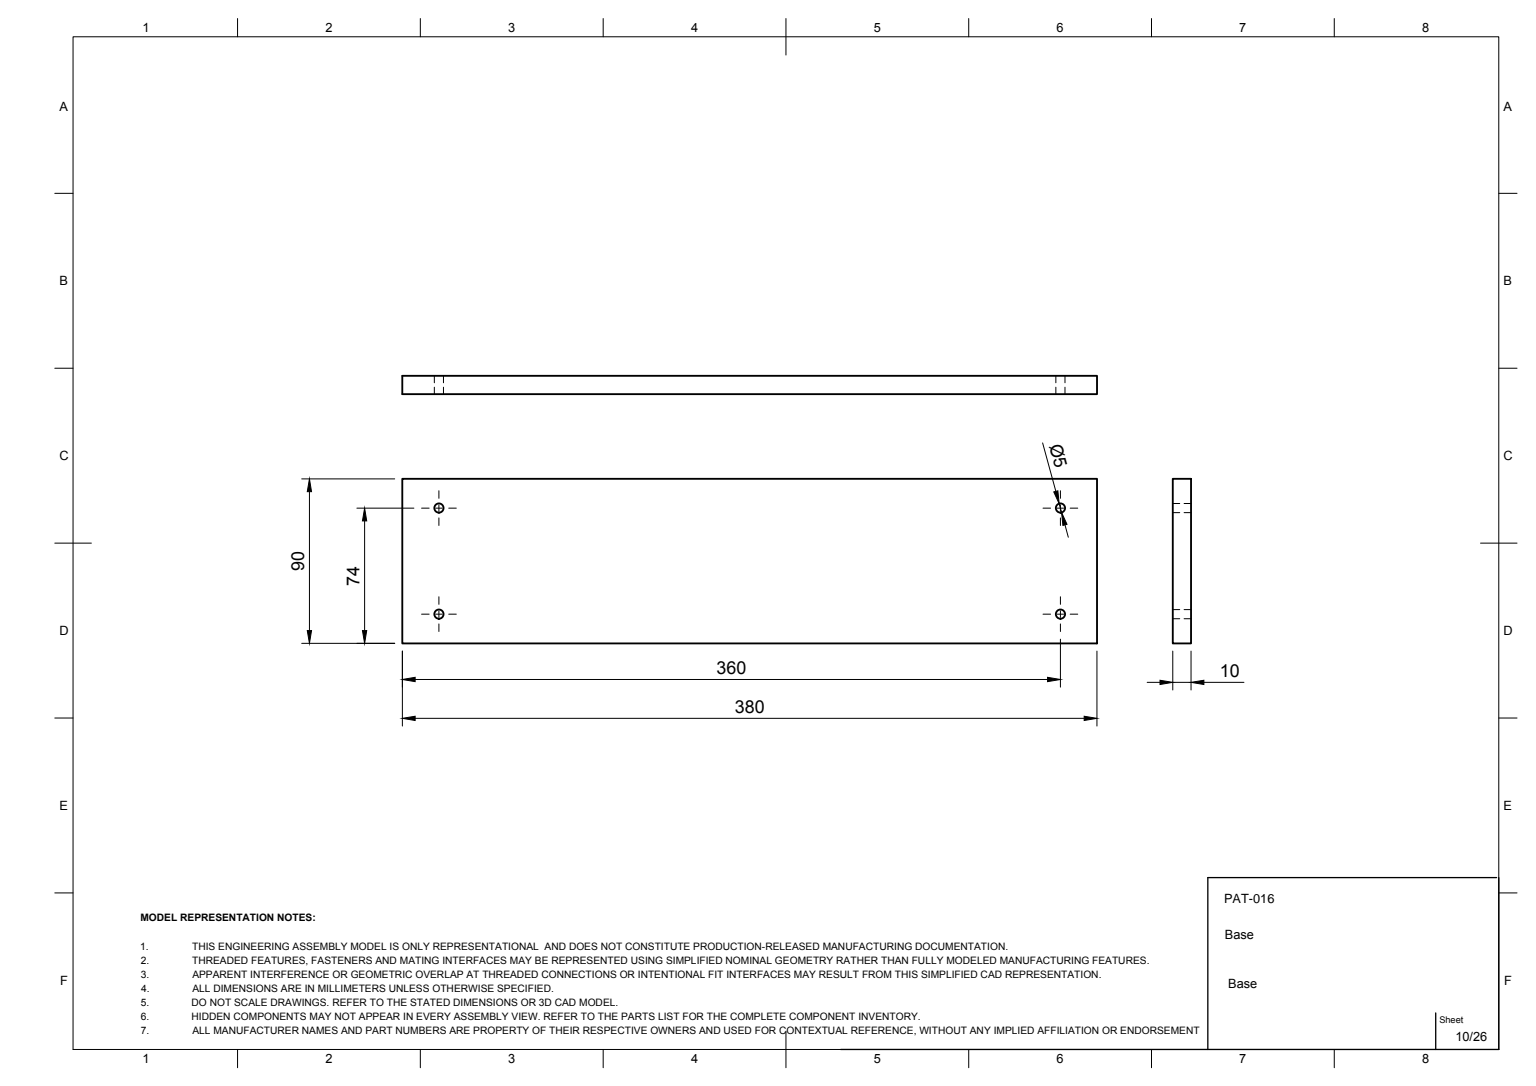
ISO-10303-21;
HEADER;
/* Generated by software containing ST-Developer
 * from STEP Tools, Inc. (www.steptools.com) 
 */

FILE_DESCRIPTION(
/* description */ ('Bracket-mounted idler roller'),
/* implementation_level */ '2;1');

FILE_NAME(
/* name */ 'Base.step',
/* time_stamp */ '2026-10-28T03:26:42-07:00',
/* author */ (''),
/* organization */ (''),
/* preprocessor_version */ 'ST-DEVELOPER v20.2',
/* originating_system */ 'Autodesk Translation Framework v15.17.0.0',
/* authorisation */ '');

FILE_SCHEMA (('AUTOMOTIVE_DESIGN { 1 0 10303 214 3 1 1 }'));
ENDSEC;

DATA;
#10=MECHANICAL_DESIGN_GEOMETRIC_PRESENTATION_REPRESENTATION('',(#285),#6241);
#243=SHAPE_REPRESENTATION_RELATIONSHIP('SRR','None',#6347,#264);
#264=ADVANCED_BREP_SHAPE_REPRESENTATION('',(#314),#6223);
#285=STYLED_ITEM('',(#6517),#314);
#314=MANIFOLD_SOLID_BREP('Body1',#3187);
#358=FACE_BOUND('',#785,.T.);
#359=FACE_BOUND('',#786,.T.);
#360=FACE_BOUND('',#787,.T.);
#361=FACE_BOUND('',#788,.T.);
#362=FACE_BOUND('',#790,.T.);
#363=FACE_BOUND('',#791,.T.);
#364=FACE_BOUND('',#792,.T.);
#365=FACE_BOUND('',#793,.T.);
#449=PLANE('',#3542);
#450=PLANE('',#3543);
#451=PLANE('',#3544);
#452=PLANE('',#3545);
#453=PLANE('',#3546);
#454=PLANE('',#3547);
#563=FACE_OUTER_BOUND('',#776,.T.);
#564=FACE_OUTER_BOUND('',#777,.T.);
#565=FACE_OUTER_BOUND('',#778,.T.);
#566=FACE_OUTER_BOUND('',#779,.T.);
#567=FACE_OUTER_BOUND('',#780,.T.);
#568=FACE_OUTER_BOUND('',#781,.T.);
#569=FACE_OUTER_BOUND('',#782,.T.);
#570=FACE_OUTER_BOUND('',#783,.T.);
#571=FACE_OUTER_BOUND('',#784,.T.);
#572=FACE_OUTER_BOUND('',#789,.T.);
#776=EDGE_LOOP('',(#2352,#2353,#2354,#2355));
#777=EDGE_LOOP('',(#2356,#2357,#2358,#2359));
#778=EDGE_LOOP('',(#2360,#2361,#2362,#2363));
#779=EDGE_LOOP('',(#2364,#2365,#2366,#2367));
#780=EDGE_LOOP('',(#2368,#2369,#2370,#2371));
#781=EDGE_LOOP('',(#2372,#2373,#2374,#2375));
#782=EDGE_LOOP('',(#2376,#2377,#2378,#2379));
#783=EDGE_LOOP('',(#2380,#2381,#2382,#2383));
#784=EDGE_LOOP('',(#2384,#2385,#2386,#2387));
#785=EDGE_LOOP('',(#2388));
#786=EDGE_LOOP('',(#2389));
#787=EDGE_LOOP('',(#2390));
#788=EDGE_LOOP('',(#2391));
#789=EDGE_LOOP('',(#2392,#2393,#2394,#2395));
#790=EDGE_LOOP('',(#2396));
#791=EDGE_LOOP('',(#2397));
#792=EDGE_LOOP('',(#2398));
#793=EDGE_LOOP('',(#2399));
#1042=LINE('',#5164,#1224);
#1043=LINE('',#5170,#1225);
#1044=LINE('',#5176,#1226);
#1045=LINE('',#5182,#1227);
#1046=LINE('',#5187,#1228);
#1047=LINE('',#5189,#1229);
#1048=LINE('',#5191,#1230);
#1049=LINE('',#5192,#1231);
#1050=LINE('',#5195,#1232);
#1051=LINE('',#5197,#1233);
#1052=LINE('',#5198,#1234);
#1053=LINE('',#5201,#1235);
#1054=LINE('',#5203,#1236);
#1055=LINE('',#5204,#1237);
#1056=LINE('',#5206,#1238);
#1057=LINE('',#5207,#1239);
#1224=VECTOR('',#4123,0.25);
#1225=VECTOR('',#4130,0.25);
#1226=VECTOR('',#4137,0.25);
#1227=VECTOR('',#4144,0.25);
#1228=VECTOR('',#4149,1.);
#1229=VECTOR('',#4150,1.);
#1230=VECTOR('',#4151,1.);
#1231=VECTOR('',#4152,1.);
#1232=VECTOR('',#4155,1.);
#1233=VECTOR('',#4156,1.);
#1234=VECTOR('',#4157,1.);
#1235=VECTOR('',#4160,1.);
#1236=VECTOR('',#4161,1.);
#1237=VECTOR('',#4162,1.);
#1238=VECTOR('',#4165,1.);
#1239=VECTOR('',#4166,1.);
#1373=CIRCLE('',#3531,0.25);
#1374=CIRCLE('',#3532,0.25);
#1375=CIRCLE('',#3534,0.25);
#1376=CIRCLE('',#3535,0.25);
#1377=CIRCLE('',#3537,0.25);
#1378=CIRCLE('',#3538,0.25);
#1379=CIRCLE('',#3540,0.25);
#1380=CIRCLE('',#3541,0.25);
#1586=VERTEX_POINT('',#5161);
#1587=VERTEX_POINT('',#5163);
#1588=VERTEX_POINT('',#5167);
#1589=VERTEX_POINT('',#5169);
#1590=VERTEX_POINT('',#5173);
#1591=VERTEX_POINT('',#5175);
#1592=VERTEX_POINT('',#5179);
#1593=VERTEX_POINT('',#5181);
#1594=VERTEX_POINT('',#5185);
#1595=VERTEX_POINT('',#5186);
#1596=VERTEX_POINT('',#5188);
#1597=VERTEX_POINT('',#5190);
#1598=VERTEX_POINT('',#5194);
#1599=VERTEX_POINT('',#5196);
#1600=VERTEX_POINT('',#5200);
#1601=VERTEX_POINT('',#5202);
#1878=EDGE_CURVE('',#1586,#1586,#1373,.T.);
#1879=EDGE_CURVE('',#1586,#1587,#1042,.T.);
#1880=EDGE_CURVE('',#1587,#1587,#1374,.T.);
#1881=EDGE_CURVE('',#1588,#1588,#1375,.T.);
#1882=EDGE_CURVE('',#1588,#1589,#1043,.T.);
#1883=EDGE_CURVE('',#1589,#1589,#1376,.T.);
#1884=EDGE_CURVE('',#1590,#1590,#1377,.T.);
#1885=EDGE_CURVE('',#1590,#1591,#1044,.T.);
#1886=EDGE_CURVE('',#1591,#1591,#1378,.T.);
#1887=EDGE_CURVE('',#1592,#1592,#1379,.T.);
#1888=EDGE_CURVE('',#1592,#1593,#1045,.T.);
#1889=EDGE_CURVE('',#1593,#1593,#1380,.T.);
#1890=EDGE_CURVE('',#1594,#1595,#1046,.T.);
#1891=EDGE_CURVE('',#1595,#1596,#1047,.T.);
#1892=EDGE_CURVE('',#1597,#1596,#1048,.T.);
#1893=EDGE_CURVE('',#1594,#1597,#1049,.T.);
#1894=EDGE_CURVE('',#1598,#1594,#1050,.T.);
#1895=EDGE_CURVE('',#1599,#1597,#1051,.T.);
#1896=EDGE_CURVE('',#1598,#1599,#1052,.T.);
#1897=EDGE_CURVE('',#1600,#1598,#1053,.T.);
#1898=EDGE_CURVE('',#1601,#1599,#1054,.T.);
#1899=EDGE_CURVE('',#1600,#1601,#1055,.T.);
#1900=EDGE_CURVE('',#1595,#1600,#1056,.T.);
#1901=EDGE_CURVE('',#1596,#1601,#1057,.T.);
#2352=ORIENTED_EDGE('',*,*,#1878,.F.);
#2353=ORIENTED_EDGE('',*,*,#1879,.T.);
#2354=ORIENTED_EDGE('',*,*,#1880,.F.);
#2355=ORIENTED_EDGE('',*,*,#1879,.F.);
#2356=ORIENTED_EDGE('',*,*,#1881,.F.);
#2357=ORIENTED_EDGE('',*,*,#1882,.T.);
#2358=ORIENTED_EDGE('',*,*,#1883,.F.);
#2359=ORIENTED_EDGE('',*,*,#1882,.F.);
#2360=ORIENTED_EDGE('',*,*,#1884,.F.);
#2361=ORIENTED_EDGE('',*,*,#1885,.T.);
#2362=ORIENTED_EDGE('',*,*,#1886,.F.);
#2363=ORIENTED_EDGE('',*,*,#1885,.F.);
#2364=ORIENTED_EDGE('',*,*,#1887,.F.);
#2365=ORIENTED_EDGE('',*,*,#1888,.T.);
#2366=ORIENTED_EDGE('',*,*,#1889,.F.);
#2367=ORIENTED_EDGE('',*,*,#1888,.F.);
#2368=ORIENTED_EDGE('',*,*,#1890,.T.);
#2369=ORIENTED_EDGE('',*,*,#1891,.T.);
#2370=ORIENTED_EDGE('',*,*,#1892,.F.);
#2371=ORIENTED_EDGE('',*,*,#1893,.F.);
#2372=ORIENTED_EDGE('',*,*,#1894,.T.);
#2373=ORIENTED_EDGE('',*,*,#1893,.T.);
#2374=ORIENTED_EDGE('',*,*,#1895,.F.);
#2375=ORIENTED_EDGE('',*,*,#1896,.F.);
#2376=ORIENTED_EDGE('',*,*,#1897,.T.);
#2377=ORIENTED_EDGE('',*,*,#1896,.T.);
#2378=ORIENTED_EDGE('',*,*,#1898,.F.);
#2379=ORIENTED_EDGE('',*,*,#1899,.F.);
#2380=ORIENTED_EDGE('',*,*,#1900,.T.);
#2381=ORIENTED_EDGE('',*,*,#1899,.T.);
#2382=ORIENTED_EDGE('',*,*,#1901,.F.);
#2383=ORIENTED_EDGE('',*,*,#1891,.F.);
#2384=ORIENTED_EDGE('',*,*,#1901,.T.);
#2385=ORIENTED_EDGE('',*,*,#1898,.T.);
#2386=ORIENTED_EDGE('',*,*,#1895,.T.);
#2387=ORIENTED_EDGE('',*,*,#1892,.T.);
#2388=ORIENTED_EDGE('',*,*,#1880,.T.);
#2389=ORIENTED_EDGE('',*,*,#1883,.T.);
#2390=ORIENTED_EDGE('',*,*,#1886,.T.);
#2391=ORIENTED_EDGE('',*,*,#1889,.T.);
#2392=ORIENTED_EDGE('',*,*,#1900,.F.);
#2393=ORIENTED_EDGE('',*,*,#1890,.F.);
#2394=ORIENTED_EDGE('',*,*,#1894,.F.);
#2395=ORIENTED_EDGE('',*,*,#1897,.F.);
#2396=ORIENTED_EDGE('',*,*,#1878,.T.);
#2397=ORIENTED_EDGE('',*,*,#1881,.T.);
#2398=ORIENTED_EDGE('',*,*,#1884,.T.);
#2399=ORIENTED_EDGE('',*,*,#1887,.T.);
#2943=CYLINDRICAL_SURFACE('',#3530,0.25);
#2944=CYLINDRICAL_SURFACE('',#3533,0.25);
#2945=CYLINDRICAL_SURFACE('',#3536,0.25);
#2946=CYLINDRICAL_SURFACE('',#3539,0.25);
#3038=ADVANCED_FACE('',(#563),#2943,.F.);
#3039=ADVANCED_FACE('',(#564),#2944,.F.);
#3040=ADVANCED_FACE('',(#565),#2945,.F.);
#3041=ADVANCED_FACE('',(#566),#2946,.F.);
#3042=ADVANCED_FACE('',(#567),#449,.T.);
#3043=ADVANCED_FACE('',(#568),#450,.T.);
#3044=ADVANCED_FACE('',(#569),#451,.T.);
#3045=ADVANCED_FACE('',(#570),#452,.T.);
#3046=ADVANCED_FACE('',(#571,#358,#359,#360,#361),#453,.T.);
#3047=ADVANCED_FACE('',(#572,#362,#363,#364,#365),#454,.F.);
#3187=CLOSED_SHELL('',(#3038,#3039,#3040,#3041,#3042,#3043,#3044,#3045,
#3046,#3047));
#3529=AXIS2_PLACEMENT_3D('',#5159,#4117,#4118);
#3530=AXIS2_PLACEMENT_3D('',#5160,#4119,#4120);
#3531=AXIS2_PLACEMENT_3D('',#5162,#4121,#4122);
#3532=AXIS2_PLACEMENT_3D('',#5165,#4124,#4125);
#3533=AXIS2_PLACEMENT_3D('',#5166,#4126,#4127);
#3534=AXIS2_PLACEMENT_3D('',#5168,#4128,#4129);
#3535=AXIS2_PLACEMENT_3D('',#5171,#4131,#4132);
#3536=AXIS2_PLACEMENT_3D('',#5172,#4133,#4134);
#3537=AXIS2_PLACEMENT_3D('',#5174,#4135,#4136);
#3538=AXIS2_PLACEMENT_3D('',#5177,#4138,#4139);
#3539=AXIS2_PLACEMENT_3D('',#5178,#4140,#4141);
#3540=AXIS2_PLACEMENT_3D('',#5180,#4142,#4143);
#3541=AXIS2_PLACEMENT_3D('',#5183,#4145,#4146);
#3542=AXIS2_PLACEMENT_3D('',#5184,#4147,#4148);
#3543=AXIS2_PLACEMENT_3D('',#5193,#4153,#4154);
#3544=AXIS2_PLACEMENT_3D('',#5199,#4158,#4159);
#3545=AXIS2_PLACEMENT_3D('',#5205,#4163,#4164);
#3546=AXIS2_PLACEMENT_3D('',#5208,#4167,#4168);
#3547=AXIS2_PLACEMENT_3D('',#5209,#4169,#4170);
#4117=DIRECTION('axis',(0.,0.,1.));
#4118=DIRECTION('refdir',(1.,0.,0.));
#4119=DIRECTION('center_axis',(0.,0.,1.));
#4120=DIRECTION('ref_axis',(1.,0.,0.));
#4121=DIRECTION('center_axis',(0.,0.,1.));
#4122=DIRECTION('ref_axis',(1.,0.,0.));
#4123=DIRECTION('',(0.,0.,1.));
#4124=DIRECTION('center_axis',(0.,0.,-1.));
#4125=DIRECTION('ref_axis',(1.,0.,0.));
#4126=DIRECTION('center_axis',(0.,0.,1.));
#4127=DIRECTION('ref_axis',(1.,0.,0.));
#4128=DIRECTION('center_axis',(0.,0.,1.));
#4129=DIRECTION('ref_axis',(1.,0.,0.));
#4130=DIRECTION('',(0.,0.,1.));
#4131=DIRECTION('center_axis',(0.,0.,-1.));
#4132=DIRECTION('ref_axis',(1.,0.,0.));
#4133=DIRECTION('center_axis',(0.,0.,1.));
#4134=DIRECTION('ref_axis',(1.,0.,0.));
#4135=DIRECTION('center_axis',(0.,0.,1.));
#4136=DIRECTION('ref_axis',(1.,0.,0.));
#4137=DIRECTION('',(0.,0.,1.));
#4138=DIRECTION('center_axis',(0.,0.,-1.));
#4139=DIRECTION('ref_axis',(1.,0.,0.));
#4140=DIRECTION('center_axis',(0.,0.,1.));
#4141=DIRECTION('ref_axis',(1.,0.,0.));
#4142=DIRECTION('center_axis',(0.,0.,1.));
#4143=DIRECTION('ref_axis',(1.,0.,0.));
#4144=DIRECTION('',(0.,0.,1.));
#4145=DIRECTION('center_axis',(0.,0.,-1.));
#4146=DIRECTION('ref_axis',(1.,0.,0.));
#4147=DIRECTION('center_axis',(0.,1.,0.));
#4148=DIRECTION('ref_axis',(-1.,0.,0.));
#4149=DIRECTION('',(-1.,0.,0.));
#4150=DIRECTION('',(0.,0.,1.));
#4151=DIRECTION('',(-1.,0.,0.));
#4152=DIRECTION('',(0.,0.,1.));
#4153=DIRECTION('center_axis',(1.,0.,0.));
#4154=DIRECTION('ref_axis',(0.,1.,0.));
#4155=DIRECTION('',(0.,1.,0.));
#4156=DIRECTION('',(0.,1.,0.));
#4157=DIRECTION('',(0.,0.,1.));
#4158=DIRECTION('center_axis',(0.,-1.,0.));
#4159=DIRECTION('ref_axis',(1.,0.,0.));
#4160=DIRECTION('',(1.,0.,0.));
#4161=DIRECTION('',(1.,0.,0.));
#4162=DIRECTION('',(0.,0.,1.));
#4163=DIRECTION('center_axis',(-1.,0.,0.));
#4164=DIRECTION('ref_axis',(0.,-1.,0.));
#4165=DIRECTION('',(0.,-1.,0.));
#4166=DIRECTION('',(0.,-1.,0.));
#4167=DIRECTION('center_axis',(0.,0.,1.));
#4168=DIRECTION('ref_axis',(1.,0.,0.));
#4169=DIRECTION('center_axis',(0.,0.,1.));
#4170=DIRECTION('ref_axis',(1.,0.,0.));
#5159=CARTESIAN_POINT('',(0.,0.,0.));
#5160=CARTESIAN_POINT('Origin',(2.9,-2.,-0.1));
#5161=CARTESIAN_POINT('',(2.65,-2.,0.));
#5162=CARTESIAN_POINT('Origin',(2.9,-2.,0.));
#5163=CARTESIAN_POINT('',(2.65,-2.,1.));
#5164=CARTESIAN_POINT('',(2.65,-2.,-0.1));
#5165=CARTESIAN_POINT('Origin',(2.9,-2.,1.));
#5166=CARTESIAN_POINT('Origin',(-2.9,32.,-0.1));
#5167=CARTESIAN_POINT('',(-3.15,32.,0.));
#5168=CARTESIAN_POINT('Origin',(-2.9,32.,0.));
#5169=CARTESIAN_POINT('',(-3.15,32.,1.));
#5170=CARTESIAN_POINT('',(-3.15,32.,-0.1));
#5171=CARTESIAN_POINT('Origin',(-2.9,32.,1.));
#5172=CARTESIAN_POINT('Origin',(-2.9,-2.,-0.1));
#5173=CARTESIAN_POINT('',(-3.15,-2.,0.));
#5174=CARTESIAN_POINT('Origin',(-2.9,-2.,0.));
#5175=CARTESIAN_POINT('',(-3.15,-2.,1.));
#5176=CARTESIAN_POINT('',(-3.15,-2.,-0.1));
#5177=CARTESIAN_POINT('Origin',(-2.9,-2.,1.));
#5178=CARTESIAN_POINT('Origin',(2.9,32.,-0.1));
#5179=CARTESIAN_POINT('',(2.65,32.,0.));
#5180=CARTESIAN_POINT('Origin',(2.9,32.,0.));
#5181=CARTESIAN_POINT('',(2.65,32.,1.));
#5182=CARTESIAN_POINT('',(2.65,32.,-0.1));
#5183=CARTESIAN_POINT('Origin',(2.9,32.,1.));
#5184=CARTESIAN_POINT('Origin',(4.5,34.,0.));
#5185=CARTESIAN_POINT('',(4.5,34.,0.));
#5186=CARTESIAN_POINT('',(-4.5,34.,0.));
#5187=CARTESIAN_POINT('',(4.5,34.,0.));
#5188=CARTESIAN_POINT('',(-4.5,34.,1.));
#5189=CARTESIAN_POINT('',(-4.5,34.,0.));
#5190=CARTESIAN_POINT('',(4.5,34.,1.));
#5191=CARTESIAN_POINT('',(4.5,34.,1.));
#5192=CARTESIAN_POINT('',(4.5,34.,0.));
#5193=CARTESIAN_POINT('Origin',(4.5,-4.,0.));
#5194=CARTESIAN_POINT('',(4.5,-4.,0.));
#5195=CARTESIAN_POINT('',(4.5,-4.,0.));
#5196=CARTESIAN_POINT('',(4.5,-4.,1.));
#5197=CARTESIAN_POINT('',(4.5,-4.,1.));
#5198=CARTESIAN_POINT('',(4.5,-4.,0.));
#5199=CARTESIAN_POINT('Origin',(-4.5,-4.,0.));
#5200=CARTESIAN_POINT('',(-4.5,-4.,0.));
#5201=CARTESIAN_POINT('',(-4.5,-4.,0.));
#5202=CARTESIAN_POINT('',(-4.5,-4.,1.));
#5203=CARTESIAN_POINT('',(-4.5,-4.,1.));
#5204=CARTESIAN_POINT('',(-4.5,-4.,0.));
#5205=CARTESIAN_POINT('Origin',(-4.5,34.,0.));
#5206=CARTESIAN_POINT('',(-4.5,34.,0.));
#5207=CARTESIAN_POINT('',(-4.5,34.,1.));
#5208=CARTESIAN_POINT('Origin',(0.,15.,1.));
#5209=CARTESIAN_POINT('Origin',(0.,15.,0.));
#6197=UNCERTAINTY_MEASURE_WITH_UNIT(LENGTH_MEASURE(0.001),#6242,
'DISTANCE_ACCURACY_VALUE',
'Maximum model space distance between geometric entities at asserted c
onnectivities');
#6215=UNCERTAINTY_MEASURE_WITH_UNIT(LENGTH_MEASURE(0.001),#6242,
'DISTANCE_ACCURACY_VALUE',
'Maximum model space distance between geometric entities at asserted c
onnectivities');
#6223=(
GEOMETRIC_REPRESENTATION_CONTEXT(3)
GLOBAL_UNCERTAINTY_ASSIGNED_CONTEXT((#6197))
GLOBAL_UNIT_ASSIGNED_CONTEXT((#6242,#6244,#6245))
REPRESENTATION_CONTEXT('','3D')
);
#6241=(
GEOMETRIC_REPRESENTATION_CONTEXT(3)
GLOBAL_UNCERTAINTY_ASSIGNED_CONTEXT((#6215))
GLOBAL_UNIT_ASSIGNED_CONTEXT((#6242,#6244,#6245))
REPRESENTATION_CONTEXT('','3D')
);
#6242=(
LENGTH_UNIT()
NAMED_UNIT(*)
SI_UNIT(.CENTI.,.METRE.)
);
#6244=(
NAMED_UNIT(*)
PLANE_ANGLE_UNIT()
SI_UNIT($,.RADIAN.)
);
#6245=(
NAMED_UNIT(*)
SI_UNIT($,.STERADIAN.)
SOLID_ANGLE_UNIT()
);
#6253=SHAPE_DEFINITION_REPRESENTATION(#6278,#6347);
#6278=PRODUCT_DEFINITION_SHAPE('',$,#6373);
#6347=SHAPE_REPRESENTATION('',(#3529),#6223);
#6365=PRODUCT_DEFINITION_CONTEXT('part definition',#6442,'design');
#6373=PRODUCT_DEFINITION('Base','Base',#6398,#6365);
#6398=PRODUCT_DEFINITION_FORMATION('',$,#6451);
#6442=APPLICATION_CONTEXT(
'Core Data for Automotive Mechanical Design Process');
#6443=PRODUCT_CONTEXT('part definition',#6442,'mechanical');
#6451=PRODUCT('Base','Base','Base',(#6443));
#6511=COLOUR_RGB('Dark Blue',0.08,0.2,0.34);
#6512=FILL_AREA_STYLE_COLOUR('',#6511);
#6513=FILL_AREA_STYLE('',(#6512));
#6514=SURFACE_STYLE_FILL_AREA(#6513);
#6515=SURFACE_SIDE_STYLE('',(#6514));
#6516=SURFACE_STYLE_USAGE(.BOTH.,#6515);
#6517=PRESENTATION_STYLE_ASSIGNMENT((#6516));
ENDSEC;
END-ISO-10303-21;
